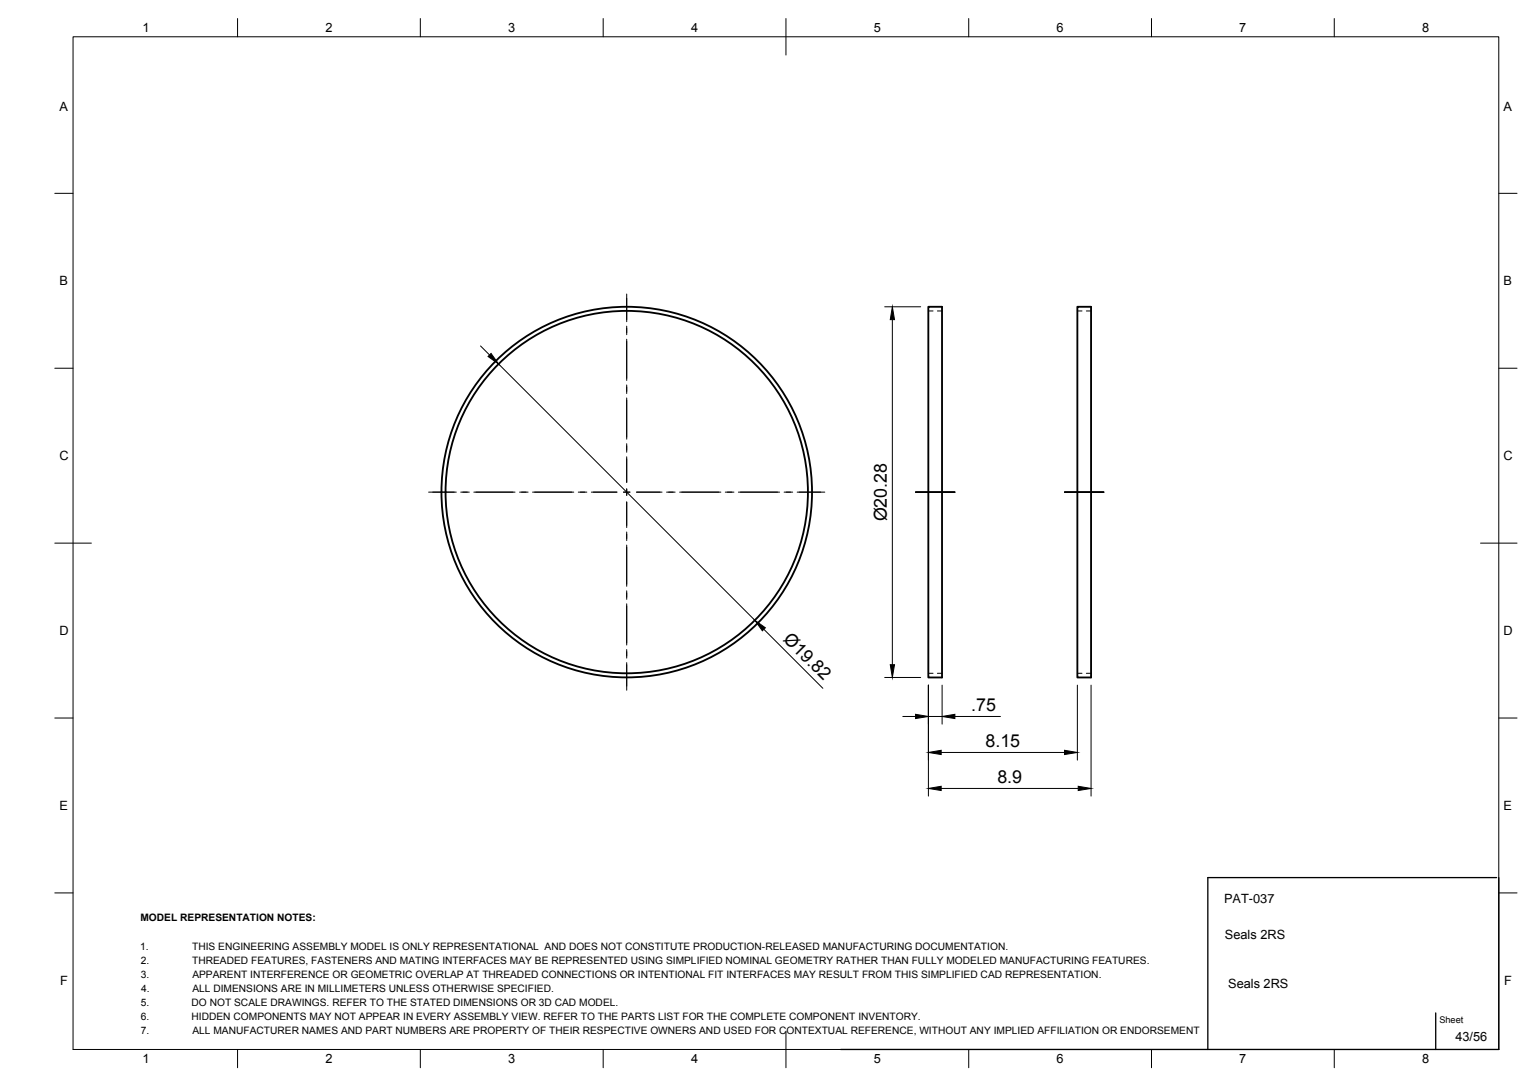
ISO-10303-21;
HEADER;
/* Generated by software containing ST-Developer
 * from STEP Tools, Inc. (www.steptools.com) 
 */

FILE_DESCRIPTION(
/* description */ ('Flywheel Crank-Slider'),
/* implementation_level */ '2;1');

FILE_NAME(
/* name */ 'Seals 2RS.step',
/* time_stamp */ '2026-10-28T03:23:13-07:00',
/* author */ (''),
/* organization */ (''),
/* preprocessor_version */ 'ST-DEVELOPER v20.2',
/* originating_system */ 'Autodesk Translation Framework v15.17.0.0',
/* authorisation */ '');

FILE_SCHEMA (('AUTOMOTIVE_DESIGN { 1 0 10303 214 3 1 1 }'));
ENDSEC;

DATA;
#10=MECHANICAL_DESIGN_GEOMETRIC_PRESENTATION_REPRESENTATION('',(#717,#718),#17322);
#605=SHAPE_REPRESENTATION_RELATIONSHIP('SRR','None',#17605,#657);
#657=ADVANCED_BREP_SHAPE_REPRESENTATION('',(#774,#775),#17309);
#717=STYLED_ITEM('',(#17931),#774);
#718=STYLED_ITEM('',(#17931),#775);
#774=MANIFOLD_SOLID_BREP('Body1',#9099);
#775=MANIFOLD_SOLID_BREP('Body2',#9100);
#948=FACE_BOUND('',#2444,.T.);
#949=FACE_BOUND('',#2447,.T.);
#950=FACE_BOUND('',#2450,.T.);
#951=FACE_BOUND('',#2453,.T.);
#1255=PLANE('',#10506);
#1256=PLANE('',#10511);
#1257=PLANE('',#10514);
#1258=PLANE('',#10519);
#1745=FACE_OUTER_BOUND('',#2443,.T.);
#1746=FACE_OUTER_BOUND('',#2445,.T.);
#1747=FACE_OUTER_BOUND('',#2446,.T.);
#1748=FACE_OUTER_BOUND('',#2448,.T.);
#1749=FACE_OUTER_BOUND('',#2449,.T.);
#1750=FACE_OUTER_BOUND('',#2451,.T.);
#1751=FACE_OUTER_BOUND('',#2452,.T.);
#1752=FACE_OUTER_BOUND('',#2454,.T.);
#2443=EDGE_LOOP('',(#7886));
#2444=EDGE_LOOP('',(#7887));
#2445=EDGE_LOOP('',(#7888,#7889,#7890,#7891));
#2446=EDGE_LOOP('',(#7892));
#2447=EDGE_LOOP('',(#7893));
#2448=EDGE_LOOP('',(#7894,#7895,#7896,#7897));
#2449=EDGE_LOOP('',(#7898));
#2450=EDGE_LOOP('',(#7899));
#2451=EDGE_LOOP('',(#7900,#7901,#7902,#7903));
#2452=EDGE_LOOP('',(#7904));
#2453=EDGE_LOOP('',(#7905));
#2454=EDGE_LOOP('',(#7906,#7907,#7908,#7909));
#3098=LINE('',#16609,#3709);
#3099=LINE('',#16614,#3710);
#3100=LINE('',#16623,#3711);
#3101=LINE('',#16628,#3712);
#3709=VECTOR('',#12964,1.013815);
#3710=VECTOR('',#12971,0.991185);
#3711=VECTOR('',#12982,1.013815);
#3712=VECTOR('',#12989,0.991185);
#4184=CIRCLE('',#10507,1.013815);
#4185=CIRCLE('',#10508,0.991185);
#4186=CIRCLE('',#10510,1.013815);
#4187=CIRCLE('',#10512,0.991185);
#4188=CIRCLE('',#10515,1.013815);
#4189=CIRCLE('',#10516,0.991185);
#4190=CIRCLE('',#10518,1.013815);
#4191=CIRCLE('',#10520,0.991185);
#4871=VERTEX_POINT('',#16602);
#4872=VERTEX_POINT('',#16604);
#4873=VERTEX_POINT('',#16607);
#4874=VERTEX_POINT('',#16611);
#4875=VERTEX_POINT('',#16616);
#4876=VERTEX_POINT('',#16618);
#4877=VERTEX_POINT('',#16621);
#4878=VERTEX_POINT('',#16625);
#5900=EDGE_CURVE('',#4871,#4871,#4184,.T.);
#5901=EDGE_CURVE('',#4872,#4872,#4185,.T.);
#5902=EDGE_CURVE('',#4873,#4873,#4186,.T.);
#5903=EDGE_CURVE('',#4873,#4871,#3098,.T.);
#5904=EDGE_CURVE('',#4874,#4874,#4187,.T.);
#5905=EDGE_CURVE('',#4874,#4872,#3099,.T.);
#5906=EDGE_CURVE('',#4875,#4875,#4188,.T.);
#5907=EDGE_CURVE('',#4876,#4876,#4189,.T.);
#5908=EDGE_CURVE('',#4877,#4877,#4190,.T.);
#5909=EDGE_CURVE('',#4877,#4875,#3100,.T.);
#5910=EDGE_CURVE('',#4878,#4878,#4191,.T.);
#5911=EDGE_CURVE('',#4878,#4876,#3101,.T.);
#7886=ORIENTED_EDGE('',*,*,#5900,.F.);
#7887=ORIENTED_EDGE('',*,*,#5901,.T.);
#7888=ORIENTED_EDGE('',*,*,#5902,.F.);
#7889=ORIENTED_EDGE('',*,*,#5903,.T.);
#7890=ORIENTED_EDGE('',*,*,#5900,.T.);
#7891=ORIENTED_EDGE('',*,*,#5903,.F.);
#7892=ORIENTED_EDGE('',*,*,#5902,.T.);
#7893=ORIENTED_EDGE('',*,*,#5904,.F.);
#7894=ORIENTED_EDGE('',*,*,#5904,.T.);
#7895=ORIENTED_EDGE('',*,*,#5905,.T.);
#7896=ORIENTED_EDGE('',*,*,#5901,.F.);
#7897=ORIENTED_EDGE('',*,*,#5905,.F.);
#7898=ORIENTED_EDGE('',*,*,#5906,.F.);
#7899=ORIENTED_EDGE('',*,*,#5907,.T.);
#7900=ORIENTED_EDGE('',*,*,#5908,.F.);
#7901=ORIENTED_EDGE('',*,*,#5909,.T.);
#7902=ORIENTED_EDGE('',*,*,#5906,.T.);
#7903=ORIENTED_EDGE('',*,*,#5909,.F.);
#7904=ORIENTED_EDGE('',*,*,#5908,.T.);
#7905=ORIENTED_EDGE('',*,*,#5910,.F.);
#7906=ORIENTED_EDGE('',*,*,#5910,.T.);
#7907=ORIENTED_EDGE('',*,*,#5911,.T.);
#7908=ORIENTED_EDGE('',*,*,#5907,.F.);
#7909=ORIENTED_EDGE('',*,*,#5911,.F.);
#8469=CYLINDRICAL_SURFACE('',#10509,1.013815);
#8470=CYLINDRICAL_SURFACE('',#10513,0.991185);
#8471=CYLINDRICAL_SURFACE('',#10517,1.013815);
#8472=CYLINDRICAL_SURFACE('',#10521,0.991185);
#8936=ADVANCED_FACE('',(#1745,#948),#1255,.T.);
#8937=ADVANCED_FACE('',(#1746),#8469,.T.);
#8938=ADVANCED_FACE('',(#1747,#949),#1256,.T.);
#8939=ADVANCED_FACE('',(#1748),#8470,.F.);
#8940=ADVANCED_FACE('',(#1749,#950),#1257,.T.);
#8941=ADVANCED_FACE('',(#1750),#8471,.T.);
#8942=ADVANCED_FACE('',(#1751,#951),#1258,.T.);
#8943=ADVANCED_FACE('',(#1752),#8472,.F.);
#9099=CLOSED_SHELL('',(#8936,#8937,#8938,#8939));
#9100=CLOSED_SHELL('',(#8940,#8941,#8942,#8943));
#10505=AXIS2_PLACEMENT_3D('',#16600,#12952,#12953);
#10506=AXIS2_PLACEMENT_3D('',#16601,#12954,#12955);
#10507=AXIS2_PLACEMENT_3D('',#16603,#12956,#12957);
#10508=AXIS2_PLACEMENT_3D('',#16605,#12958,#12959);
#10509=AXIS2_PLACEMENT_3D('',#16606,#12960,#12961);
#10510=AXIS2_PLACEMENT_3D('',#16608,#12962,#12963);
#10511=AXIS2_PLACEMENT_3D('',#16610,#12965,#12966);
#10512=AXIS2_PLACEMENT_3D('',#16612,#12967,#12968);
#10513=AXIS2_PLACEMENT_3D('',#16613,#12969,#12970);
#10514=AXIS2_PLACEMENT_3D('',#16615,#12972,#12973);
#10515=AXIS2_PLACEMENT_3D('',#16617,#12974,#12975);
#10516=AXIS2_PLACEMENT_3D('',#16619,#12976,#12977);
#10517=AXIS2_PLACEMENT_3D('',#16620,#12978,#12979);
#10518=AXIS2_PLACEMENT_3D('',#16622,#12980,#12981);
#10519=AXIS2_PLACEMENT_3D('',#16624,#12983,#12984);
#10520=AXIS2_PLACEMENT_3D('',#16626,#12985,#12986);
#10521=AXIS2_PLACEMENT_3D('',#16627,#12987,#12988);
#12952=DIRECTION('axis',(0.,0.,1.));
#12953=DIRECTION('refdir',(1.,0.,0.));
#12954=DIRECTION('center_axis',(0.,1.,0.));
#12955=DIRECTION('ref_axis',(0.,0.,1.));
#12956=DIRECTION('center_axis',(0.,-1.,0.));
#12957=DIRECTION('ref_axis',(1.,0.,0.));
#12958=DIRECTION('center_axis',(0.,-1.,0.));
#12959=DIRECTION('ref_axis',(1.,0.,0.));
#12960=DIRECTION('center_axis',(0.,-1.,0.));
#12961=DIRECTION('ref_axis',(1.,0.,0.));
#12962=DIRECTION('center_axis',(0.,-1.,0.));
#12963=DIRECTION('ref_axis',(1.,0.,0.));
#12964=DIRECTION('',(0.,1.,0.));
#12965=DIRECTION('center_axis',(0.,-1.,0.));
#12966=DIRECTION('ref_axis',(0.,0.,-1.));
#12967=DIRECTION('center_axis',(0.,-1.,0.));
#12968=DIRECTION('ref_axis',(1.,0.,0.));
#12969=DIRECTION('center_axis',(0.,-1.,0.));
#12970=DIRECTION('ref_axis',(1.,0.,0.));
#12971=DIRECTION('',(0.,1.,0.));
#12972=DIRECTION('center_axis',(0.,1.,0.));
#12973=DIRECTION('ref_axis',(0.,0.,1.));
#12974=DIRECTION('center_axis',(0.,-1.,0.));
#12975=DIRECTION('ref_axis',(1.,0.,0.));
#12976=DIRECTION('center_axis',(0.,-1.,0.));
#12977=DIRECTION('ref_axis',(1.,0.,0.));
#12978=DIRECTION('center_axis',(0.,-1.,0.));
#12979=DIRECTION('ref_axis',(1.,0.,0.));
#12980=DIRECTION('center_axis',(0.,-1.,0.));
#12981=DIRECTION('ref_axis',(1.,0.,0.));
#12982=DIRECTION('',(0.,1.,0.));
#12983=DIRECTION('center_axis',(0.,-1.,0.));
#12984=DIRECTION('ref_axis',(0.,0.,-1.));
#12985=DIRECTION('center_axis',(0.,-1.,0.));
#12986=DIRECTION('ref_axis',(1.,0.,0.));
#12987=DIRECTION('center_axis',(0.,-1.,0.));
#12988=DIRECTION('ref_axis',(1.,0.,0.));
#12989=DIRECTION('',(0.,1.,0.));
#16600=CARTESIAN_POINT('',(0.,0.,0.));
#16601=CARTESIAN_POINT('Origin',(1.013815,0.445,0.));
#16602=CARTESIAN_POINT('',(-1.013815,0.445,-1.24156529467757E-16));
#16603=CARTESIAN_POINT('Origin',(0.,0.445,0.));
#16604=CARTESIAN_POINT('',(-0.991185,0.445,-1.21385153761287E-16));
#16605=CARTESIAN_POINT('Origin',(0.,0.445,0.));
#16606=CARTESIAN_POINT('Origin',(0.,0.4075,0.));
#16607=CARTESIAN_POINT('',(-1.013815,0.37,-1.24156529467757E-16));
#16608=CARTESIAN_POINT('Origin',(0.,0.37,0.));
#16609=CARTESIAN_POINT('',(-1.013815,0.4075,-1.24156529467757E-16));
#16610=CARTESIAN_POINT('Origin',(0.991185,0.37,0.));
#16611=CARTESIAN_POINT('',(-0.991185,0.37,-1.21385153761287E-16));
#16612=CARTESIAN_POINT('Origin',(0.,0.37,0.));
#16613=CARTESIAN_POINT('Origin',(0.,0.4075,0.));
#16614=CARTESIAN_POINT('',(-0.991185,0.4075,-1.21385153761287E-16));
#16615=CARTESIAN_POINT('Origin',(1.013815,-0.37,0.));
#16616=CARTESIAN_POINT('',(-1.013815,-0.37,-1.24156529467757E-16));
#16617=CARTESIAN_POINT('Origin',(0.,-0.37,0.));
#16618=CARTESIAN_POINT('',(-0.991185,-0.37,-1.21385153761287E-16));
#16619=CARTESIAN_POINT('Origin',(0.,-0.37,0.));
#16620=CARTESIAN_POINT('Origin',(0.,-0.4075,0.));
#16621=CARTESIAN_POINT('',(-1.013815,-0.445,-1.24156529467757E-16));
#16622=CARTESIAN_POINT('Origin',(0.,-0.445,0.));
#16623=CARTESIAN_POINT('',(-1.013815,-0.4075,-1.24156529467757E-16));
#16624=CARTESIAN_POINT('Origin',(0.991185,-0.445,0.));
#16625=CARTESIAN_POINT('',(-0.991185,-0.445,-1.21385153761287E-16));
#16626=CARTESIAN_POINT('Origin',(0.,-0.445,0.));
#16627=CARTESIAN_POINT('Origin',(0.,-0.4075,0.));
#16628=CARTESIAN_POINT('',(-0.991185,-0.4075,-1.21385153761287E-16));
#17248=UNCERTAINTY_MEASURE_WITH_UNIT(LENGTH_MEASURE(0.001),#17323,
'DISTANCE_ACCURACY_VALUE',
'Maximum model space distance between geometric entities at asserted c
onnectivities');
#17261=UNCERTAINTY_MEASURE_WITH_UNIT(LENGTH_MEASURE(0.001),#17323,
'DISTANCE_ACCURACY_VALUE',
'Maximum model space distance between geometric entities at asserted c
onnectivities');
#17309=(
GEOMETRIC_REPRESENTATION_CONTEXT(3)
GLOBAL_UNCERTAINTY_ASSIGNED_CONTEXT((#17248))
GLOBAL_UNIT_ASSIGNED_CONTEXT((#17323,#17325,#17326))
REPRESENTATION_CONTEXT('','3D')
);
#17322=(
GEOMETRIC_REPRESENTATION_CONTEXT(3)
GLOBAL_UNCERTAINTY_ASSIGNED_CONTEXT((#17261))
GLOBAL_UNIT_ASSIGNED_CONTEXT((#17323,#17325,#17326))
REPRESENTATION_CONTEXT('','3D')
);
#17323=(
LENGTH_UNIT()
NAMED_UNIT(*)
SI_UNIT(.CENTI.,.METRE.)
);
#17325=(
NAMED_UNIT(*)
PLANE_ANGLE_UNIT()
SI_UNIT($,.RADIAN.)
);
#17326=(
NAMED_UNIT(*)
SI_UNIT($,.STERADIAN.)
SOLID_ANGLE_UNIT()
);
#17374=SHAPE_DEFINITION_REPRESENTATION(#17436,#17605);
#17436=PRODUCT_DEFINITION_SHAPE('',$,#17666);
#17605=SHAPE_REPRESENTATION('',(#10505),#17309);
#17618=PRODUCT_DEFINITION_CONTEXT('part definition',#17800,'design');
#17666=PRODUCT_DEFINITION('Seals 2RS','Seals 2RS',#17726,#17618);
#17726=PRODUCT_DEFINITION_FORMATION('',$,#17849);
#17800=APPLICATION_CONTEXT(
'Core Data for Automotive Mechanical Design Process');
#17801=PRODUCT_CONTEXT('part definition',#17800,'mechanical');
#17849=PRODUCT('Seals 2RS','Seals 2RS','Seals 2RS',(#17801));
#17925=COLOUR_RGB('Grey',0.48,0.52,0.57);
#17926=FILL_AREA_STYLE_COLOUR('',#17925);
#17927=FILL_AREA_STYLE('',(#17926));
#17928=SURFACE_STYLE_FILL_AREA(#17927);
#17929=SURFACE_SIDE_STYLE('',(#17928));
#17930=SURFACE_STYLE_USAGE(.BOTH.,#17929);
#17931=PRESENTATION_STYLE_ASSIGNMENT((#17930));
ENDSEC;
END-ISO-10303-21;
